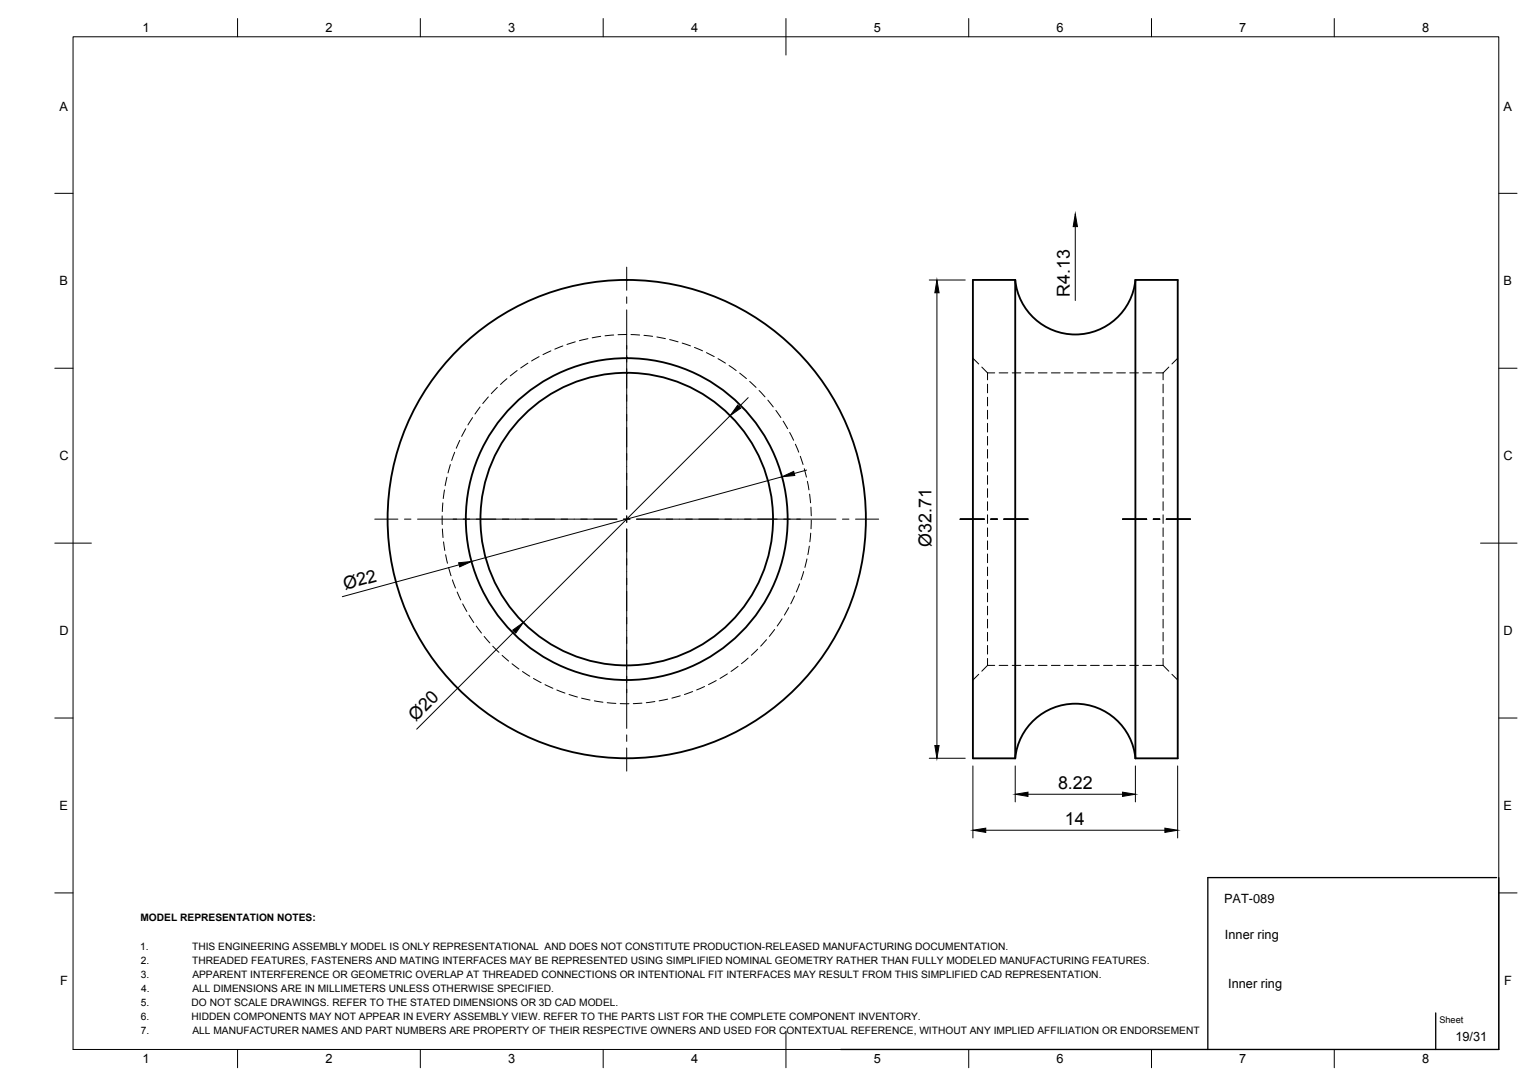
ISO-10303-21;
HEADER;
/* Generated by software containing ST-Developer
 * from STEP Tools, Inc. (www.steptools.com) 
 */

FILE_DESCRIPTION(
/* description */ ('Rotary union on bearing shaft'),
/* implementation_level */ '2;1');

FILE_NAME(
/* name */ 'Inner ring.step',
/* time_stamp */ '2026-10-28T03:24:01-07:00',
/* author */ (''),
/* organization */ (''),
/* preprocessor_version */ 'ST-DEVELOPER v20.2',
/* originating_system */ 'Autodesk Translation Framework v15.17.0.0',
/* authorisation */ '');

FILE_SCHEMA (('AUTOMOTIVE_DESIGN { 1 0 10303 214 3 1 1 }'));
ENDSEC;

DATA;
#10=MECHANICAL_DESIGN_GEOMETRIC_PRESENTATION_REPRESENTATION('',(#324),#9448);
#201=CONICAL_SURFACE('',#5440,1.05,0.785398163397449);
#202=CONICAL_SURFACE('',#5447,1.05,0.785398163397449);
#223=TOROIDAL_SURFACE('',#5429,1.675,0.412776);
#270=SHAPE_REPRESENTATION_RELATIONSHIP('SRR','None',#9571,#297);
#297=ADVANCED_BREP_SHAPE_REPRESENTATION('',(#359),#9431);
#324=STYLED_ITEM('',(#9778),#359);
#359=MANIFOLD_SOLID_BREP('Body1',#4879);
#444=FACE_BOUND('',#1135,.T.);
#445=FACE_BOUND('',#1138,.T.);
#550=PLANE('',#5442);
#551=PLANE('',#5445);
#767=FACE_OUTER_BOUND('',#1130,.T.);
#768=FACE_OUTER_BOUND('',#1131,.T.);
#769=FACE_OUTER_BOUND('',#1132,.T.);
#770=FACE_OUTER_BOUND('',#1133,.T.);
#771=FACE_OUTER_BOUND('',#1134,.T.);
#772=FACE_OUTER_BOUND('',#1136,.T.);
#773=FACE_OUTER_BOUND('',#1137,.T.);
#774=FACE_OUTER_BOUND('',#1139,.T.);
#1130=EDGE_LOOP('',(#3723,#3724,#3725,#3726,#3727,#3728));
#1131=EDGE_LOOP('',(#3729,#3730,#3731,#3732,#3733));
#1132=EDGE_LOOP('',(#3734,#3735,#3736,#3737));
#1133=EDGE_LOOP('',(#3738,#3739,#3740,#3741));
#1134=EDGE_LOOP('',(#3742));
#1135=EDGE_LOOP('',(#3743));
#1136=EDGE_LOOP('',(#3744,#3745,#3746,#3747,#3748));
#1137=EDGE_LOOP('',(#3749));
#1138=EDGE_LOOP('',(#3750));
#1139=EDGE_LOOP('',(#3751,#3752,#3753,#3754));
#1482=LINE('',#8042,#1802);
#1483=LINE('',#8048,#1803);
#1484=LINE('',#8052,#1804);
#1485=LINE('',#8058,#1805);
#1486=LINE('',#8063,#1806);
#1802=VECTOR('',#6413,1.63531);
#1803=VECTOR('',#6420,1.);
#1804=VECTOR('',#6425,1.05);
#1805=VECTOR('',#6434,1.63531);
#1806=VECTOR('',#6441,1.05);
#2100=CIRCLE('',#5430,1.63531);
#2101=CIRCLE('',#5431,1.63531);
#2102=CIRCLE('',#5432,0.412776);
#2103=CIRCLE('',#5433,1.63531);
#2104=CIRCLE('',#5434,1.63531);
#2105=CIRCLE('',#5436,1.63531);
#2106=CIRCLE('',#5438,1.);
#2107=CIRCLE('',#5439,1.);
#2108=CIRCLE('',#5441,1.1);
#2109=CIRCLE('',#5444,1.63531);
#2110=CIRCLE('',#5446,1.1);
#2404=VERTEX_POINT('',#8031);
#2405=VERTEX_POINT('',#8032);
#2406=VERTEX_POINT('',#8035);
#2407=VERTEX_POINT('',#8037);
#2408=VERTEX_POINT('',#8041);
#2409=VERTEX_POINT('',#8045);
#2410=VERTEX_POINT('',#8047);
#2411=VERTEX_POINT('',#8051);
#2412=VERTEX_POINT('',#8056);
#2413=VERTEX_POINT('',#8060);
#2889=EDGE_CURVE('',#2404,#2405,#2100,.T.);
#2890=EDGE_CURVE('',#2405,#2404,#2101,.T.);
#2891=EDGE_CURVE('',#2405,#2406,#2102,.T.);
#2892=EDGE_CURVE('',#2407,#2406,#2103,.T.);
#2893=EDGE_CURVE('',#2406,#2407,#2104,.T.);
#2894=EDGE_CURVE('',#2407,#2408,#1482,.T.);
#2895=EDGE_CURVE('',#2408,#2408,#2105,.T.);
#2896=EDGE_CURVE('',#2409,#2409,#2106,.T.);
#2897=EDGE_CURVE('',#2409,#2410,#1483,.T.);
#2898=EDGE_CURVE('',#2410,#2410,#2107,.T.);
#2899=EDGE_CURVE('',#2410,#2411,#1484,.T.);
#2900=EDGE_CURVE('',#2411,#2411,#2108,.T.);
#2901=EDGE_CURVE('',#2412,#2412,#2109,.T.);
#2902=EDGE_CURVE('',#2412,#2404,#1485,.T.);
#2903=EDGE_CURVE('',#2413,#2413,#2110,.T.);
#2904=EDGE_CURVE('',#2413,#2409,#1486,.T.);
#3723=ORIENTED_EDGE('',*,*,#2889,.F.);
#3724=ORIENTED_EDGE('',*,*,#2890,.F.);
#3725=ORIENTED_EDGE('',*,*,#2891,.T.);
#3726=ORIENTED_EDGE('',*,*,#2892,.F.);
#3727=ORIENTED_EDGE('',*,*,#2893,.F.);
#3728=ORIENTED_EDGE('',*,*,#2891,.F.);
#3729=ORIENTED_EDGE('',*,*,#2892,.T.);
#3730=ORIENTED_EDGE('',*,*,#2893,.T.);
#3731=ORIENTED_EDGE('',*,*,#2894,.T.);
#3732=ORIENTED_EDGE('',*,*,#2895,.T.);
#3733=ORIENTED_EDGE('',*,*,#2894,.F.);
#3734=ORIENTED_EDGE('',*,*,#2896,.T.);
#3735=ORIENTED_EDGE('',*,*,#2897,.T.);
#3736=ORIENTED_EDGE('',*,*,#2898,.F.);
#3737=ORIENTED_EDGE('',*,*,#2897,.F.);
#3738=ORIENTED_EDGE('',*,*,#2898,.T.);
#3739=ORIENTED_EDGE('',*,*,#2899,.T.);
#3740=ORIENTED_EDGE('',*,*,#2900,.F.);
#3741=ORIENTED_EDGE('',*,*,#2899,.F.);
#3742=ORIENTED_EDGE('',*,*,#2895,.F.);
#3743=ORIENTED_EDGE('',*,*,#2900,.T.);
#3744=ORIENTED_EDGE('',*,*,#2901,.F.);
#3745=ORIENTED_EDGE('',*,*,#2902,.T.);
#3746=ORIENTED_EDGE('',*,*,#2889,.T.);
#3747=ORIENTED_EDGE('',*,*,#2890,.T.);
#3748=ORIENTED_EDGE('',*,*,#2902,.F.);
#3749=ORIENTED_EDGE('',*,*,#2901,.T.);
#3750=ORIENTED_EDGE('',*,*,#2903,.F.);
#3751=ORIENTED_EDGE('',*,*,#2903,.T.);
#3752=ORIENTED_EDGE('',*,*,#2904,.T.);
#3753=ORIENTED_EDGE('',*,*,#2896,.F.);
#3754=ORIENTED_EDGE('',*,*,#2904,.F.);
#4525=CYLINDRICAL_SURFACE('',#5435,1.63531);
#4526=CYLINDRICAL_SURFACE('',#5437,1.);
#4527=CYLINDRICAL_SURFACE('',#5443,1.63531);
#4680=ADVANCED_FACE('',(#767),#223,.F.);
#4681=ADVANCED_FACE('',(#768),#4525,.T.);
#4682=ADVANCED_FACE('',(#769),#4526,.F.);
#4683=ADVANCED_FACE('',(#770),#201,.F.);
#4684=ADVANCED_FACE('',(#771,#444),#550,.T.);
#4685=ADVANCED_FACE('',(#772),#4527,.T.);
#4686=ADVANCED_FACE('',(#773,#445),#551,.T.);
#4687=ADVANCED_FACE('',(#774),#202,.F.);
#4879=CLOSED_SHELL('',(#4680,#4681,#4682,#4683,#4684,#4685,#4686,#4687));
#5428=AXIS2_PLACEMENT_3D('',#8029,#6397,#6398);
#5429=AXIS2_PLACEMENT_3D('',#8030,#6399,#6400);
#5430=AXIS2_PLACEMENT_3D('',#8033,#6401,#6402);
#5431=AXIS2_PLACEMENT_3D('',#8034,#6403,#6404);
#5432=AXIS2_PLACEMENT_3D('',#8036,#6405,#6406);
#5433=AXIS2_PLACEMENT_3D('',#8038,#6407,#6408);
#5434=AXIS2_PLACEMENT_3D('',#8039,#6409,#6410);
#5435=AXIS2_PLACEMENT_3D('',#8040,#6411,#6412);
#5436=AXIS2_PLACEMENT_3D('',#8043,#6414,#6415);
#5437=AXIS2_PLACEMENT_3D('',#8044,#6416,#6417);
#5438=AXIS2_PLACEMENT_3D('',#8046,#6418,#6419);
#5439=AXIS2_PLACEMENT_3D('',#8049,#6421,#6422);
#5440=AXIS2_PLACEMENT_3D('',#8050,#6423,#6424);
#5441=AXIS2_PLACEMENT_3D('',#8053,#6426,#6427);
#5442=AXIS2_PLACEMENT_3D('',#8054,#6428,#6429);
#5443=AXIS2_PLACEMENT_3D('',#8055,#6430,#6431);
#5444=AXIS2_PLACEMENT_3D('',#8057,#6432,#6433);
#5445=AXIS2_PLACEMENT_3D('',#8059,#6435,#6436);
#5446=AXIS2_PLACEMENT_3D('',#8061,#6437,#6438);
#5447=AXIS2_PLACEMENT_3D('',#8062,#6439,#6440);
#6397=DIRECTION('axis',(0.,0.,1.));
#6398=DIRECTION('refdir',(1.,0.,0.));
#6399=DIRECTION('center_axis',(0.,-1.,0.));
#6400=DIRECTION('ref_axis',(0.,0.,-1.));
#6401=DIRECTION('center_axis',(0.,-1.,0.));
#6402=DIRECTION('ref_axis',(1.,0.,0.));
#6403=DIRECTION('center_axis',(0.,-1.,0.));
#6404=DIRECTION('ref_axis',(1.,0.,0.));
#6405=DIRECTION('center_axis',(1.,0.,1.22464679914735E-16));
#6406=DIRECTION('ref_axis',(-1.22464679914735E-16,0.,1.));
#6407=DIRECTION('center_axis',(0.,1.,0.));
#6408=DIRECTION('ref_axis',(1.,0.,0.));
#6409=DIRECTION('center_axis',(0.,1.,0.));
#6410=DIRECTION('ref_axis',(1.,0.,0.));
#6411=DIRECTION('center_axis',(0.,-1.,0.));
#6412=DIRECTION('ref_axis',(1.,0.,0.));
#6413=DIRECTION('',(0.,1.,0.));
#6414=DIRECTION('center_axis',(0.,-1.,0.));
#6415=DIRECTION('ref_axis',(1.,0.,0.));
#6416=DIRECTION('center_axis',(0.,-1.,0.));
#6417=DIRECTION('ref_axis',(1.,0.,0.));
#6418=DIRECTION('center_axis',(0.,-1.,0.));
#6419=DIRECTION('ref_axis',(1.,0.,0.));
#6420=DIRECTION('',(0.,1.,0.));
#6421=DIRECTION('center_axis',(0.,-1.,0.));
#6422=DIRECTION('ref_axis',(1.,0.,0.));
#6423=DIRECTION('center_axis',(0.,1.,0.));
#6424=DIRECTION('ref_axis',(1.,0.,0.));
#6425=DIRECTION('',(-0.707106781186548,0.707106781186547,-8.65956056235494E-17));
#6426=DIRECTION('center_axis',(0.,-1.,0.));
#6427=DIRECTION('ref_axis',(1.,0.,0.));
#6428=DIRECTION('center_axis',(0.,1.,0.));
#6429=DIRECTION('ref_axis',(0.,0.,1.));
#6430=DIRECTION('center_axis',(0.,-1.,0.));
#6431=DIRECTION('ref_axis',(1.,0.,0.));
#6432=DIRECTION('center_axis',(0.,-1.,0.));
#6433=DIRECTION('ref_axis',(1.,0.,0.));
#6434=DIRECTION('',(0.,1.,0.));
#6435=DIRECTION('center_axis',(0.,-1.,0.));
#6436=DIRECTION('ref_axis',(0.,0.,-1.));
#6437=DIRECTION('center_axis',(0.,-1.,0.));
#6438=DIRECTION('ref_axis',(1.,0.,0.));
#6439=DIRECTION('center_axis',(0.,-1.,0.));
#6440=DIRECTION('ref_axis',(1.,0.,0.));
#6441=DIRECTION('',(0.707106781186548,0.707106781186547,8.65956056235494E-17));
#8029=CARTESIAN_POINT('',(0.,0.,0.));
#8030=CARTESIAN_POINT('Origin',(0.,0.,0.));
#8031=CARTESIAN_POINT('',(-1.63531,-0.410863395882378,-2.00267715711366E-16));
#8032=CARTESIAN_POINT('',(-2.00267715711366E-16,-0.410863395882378,1.63531));
#8033=CARTESIAN_POINT('Origin',(0.,-0.410863395882378,0.));
#8034=CARTESIAN_POINT('Origin',(0.,-0.410863395882378,0.));
#8035=CARTESIAN_POINT('',(-2.00267715711366E-16,0.410863395882378,1.63531));
#8036=CARTESIAN_POINT('Origin',(-2.05128338857182E-16,0.,1.675));
#8037=CARTESIAN_POINT('',(-1.63531,0.410863395882378,2.00267715711366E-16));
#8038=CARTESIAN_POINT('Origin',(0.,0.410863395882378,0.));
#8039=CARTESIAN_POINT('Origin',(0.,0.410863395882378,0.));
#8040=CARTESIAN_POINT('Origin',(0.,0.,0.));
#8041=CARTESIAN_POINT('',(-1.63531,0.7,-2.00267715711366E-16));
#8042=CARTESIAN_POINT('',(-1.63531,0.,-2.00267715711366E-16));
#8043=CARTESIAN_POINT('Origin',(0.,0.7,0.));
#8044=CARTESIAN_POINT('Origin',(0.,0.,0.));
#8045=CARTESIAN_POINT('',(-1.,-0.6,-1.22464679914735E-16));
#8046=CARTESIAN_POINT('Origin',(0.,-0.6,0.));
#8047=CARTESIAN_POINT('',(-1.,0.6,-1.22464679914735E-16));
#8048=CARTESIAN_POINT('',(-1.,0.,-1.22464679914735E-16));
#8049=CARTESIAN_POINT('Origin',(0.,0.6,0.));
#8050=CARTESIAN_POINT('Origin',(0.,0.65,0.));
#8051=CARTESIAN_POINT('',(-1.1,0.7,-1.34711147906209E-16));
#8052=CARTESIAN_POINT('',(-1.05,0.65,-1.28587913910472E-16));
#8053=CARTESIAN_POINT('Origin',(0.,0.7,0.));
#8054=CARTESIAN_POINT('Origin',(1.63531,0.7,0.));
#8055=CARTESIAN_POINT('Origin',(0.,0.,0.));
#8056=CARTESIAN_POINT('',(-1.63531,-0.7,-2.00267715711366E-16));
#8057=CARTESIAN_POINT('Origin',(0.,-0.7,0.));
#8058=CARTESIAN_POINT('',(-1.63531,0.,-2.00267715711366E-16));
#8059=CARTESIAN_POINT('Origin',(1.1,-0.7,0.));
#8060=CARTESIAN_POINT('',(-1.1,-0.7,-1.34711147906209E-16));
#8061=CARTESIAN_POINT('Origin',(0.,-0.7,0.));
#8062=CARTESIAN_POINT('Origin',(0.,-0.65,0.));
#8063=CARTESIAN_POINT('',(-1.05,-0.65,-1.28587913910472E-16));
#9399=UNCERTAINTY_MEASURE_WITH_UNIT(LENGTH_MEASURE(0.001),#9449,
'DISTANCE_ACCURACY_VALUE',
'Maximum model space distance between geometric entities at asserted c
onnectivities');
#9416=UNCERTAINTY_MEASURE_WITH_UNIT(LENGTH_MEASURE(0.001),#9449,
'DISTANCE_ACCURACY_VALUE',
'Maximum model space distance between geometric entities at asserted c
onnectivities');
#9431=(
GEOMETRIC_REPRESENTATION_CONTEXT(3)
GLOBAL_UNCERTAINTY_ASSIGNED_CONTEXT((#9399))
GLOBAL_UNIT_ASSIGNED_CONTEXT((#9449,#9451,#9452))
REPRESENTATION_CONTEXT('','3D')
);
#9448=(
GEOMETRIC_REPRESENTATION_CONTEXT(3)
GLOBAL_UNCERTAINTY_ASSIGNED_CONTEXT((#9416))
GLOBAL_UNIT_ASSIGNED_CONTEXT((#9449,#9451,#9452))
REPRESENTATION_CONTEXT('','3D')
);
#9449=(
LENGTH_UNIT()
NAMED_UNIT(*)
SI_UNIT(.CENTI.,.METRE.)
);
#9451=(
NAMED_UNIT(*)
PLANE_ANGLE_UNIT()
SI_UNIT($,.RADIAN.)
);
#9452=(
NAMED_UNIT(*)
SI_UNIT($,.STERADIAN.)
SOLID_ANGLE_UNIT()
);
#9467=SHAPE_DEFINITION_REPRESENTATION(#9498,#9571);
#9498=PRODUCT_DEFINITION_SHAPE('',$,#9603);
#9571=SHAPE_REPRESENTATION('',(#5428),#9431);
#9588=PRODUCT_DEFINITION_CONTEXT('part definition',#9683,'design');
#9603=PRODUCT_DEFINITION('Inner ring','Inner ring',#9634,#9588);
#9634=PRODUCT_DEFINITION_FORMATION('',$,#9699);
#9683=APPLICATION_CONTEXT(
'Core Data for Automotive Mechanical Design Process');
#9684=PRODUCT_CONTEXT('part definition',#9683,'mechanical');
#9699=PRODUCT('Inner ring','Inner ring','Inner ring',(#9684));
#9772=COLOUR_RGB('Grey',0.48,0.52,0.57);
#9773=FILL_AREA_STYLE_COLOUR('',#9772);
#9774=FILL_AREA_STYLE('',(#9773));
#9775=SURFACE_STYLE_FILL_AREA(#9774);
#9776=SURFACE_SIDE_STYLE('',(#9775));
#9777=SURFACE_STYLE_USAGE(.BOTH.,#9776);
#9778=PRESENTATION_STYLE_ASSIGNMENT((#9777));
ENDSEC;
END-ISO-10303-21;
